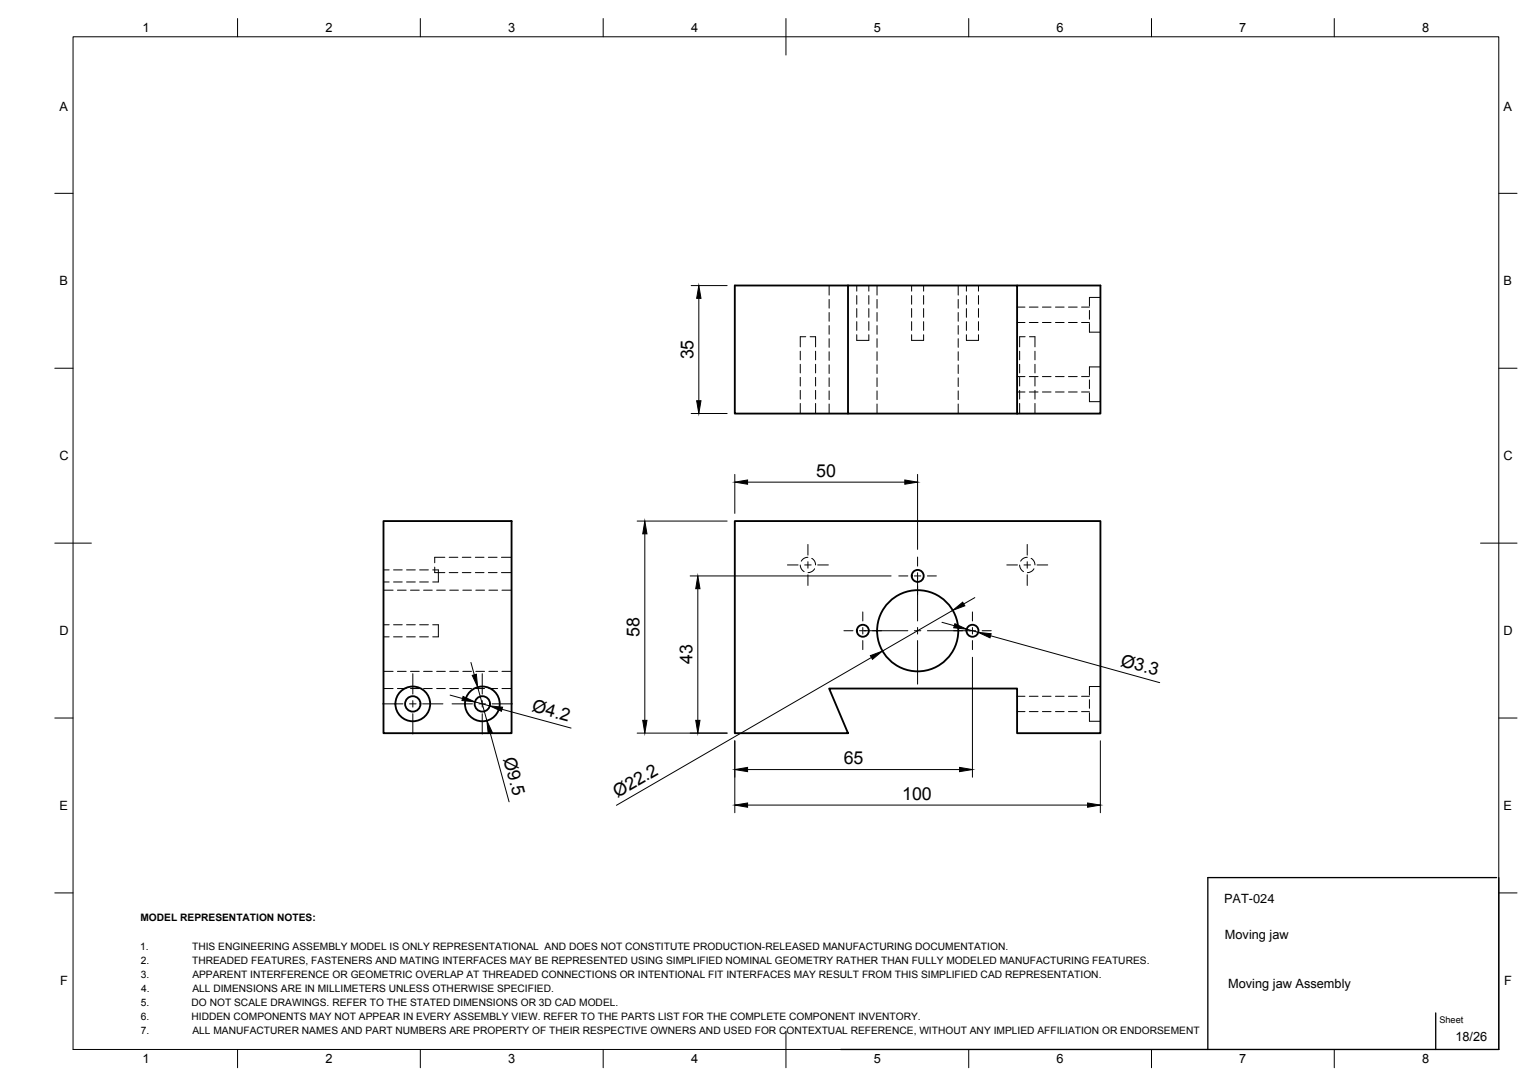
ISO-10303-21;
HEADER;
/* Generated by software containing ST-Developer
 * from STEP Tools, Inc. (www.steptools.com) 
 */

FILE_DESCRIPTION(
/* description */ ('Compact handwheel screw vise'),
/* implementation_level */ '2;1');

FILE_NAME(
/* name */ 'Moving jaw.step',
/* time_stamp */ '2026-10-29T16:08:22-07:00',
/* author */ (''),
/* organization */ (''),
/* preprocessor_version */ 'ST-DEVELOPER v20.2',
/* originating_system */ 'Autodesk Translation Framework v15.17.0.0',
/* authorisation */ '');

FILE_SCHEMA (('AUTOMOTIVE_DESIGN { 1 0 10303 214 3 1 1 }'));
ENDSEC;

DATA;
#10=MECHANICAL_DESIGN_GEOMETRIC_PRESENTATION_REPRESENTATION('',(#664),#25074);
#600=SHAPE_REPRESENTATION_RELATIONSHIP('SRR','None',#25210,#628);
#628=ADVANCED_BREP_SHAPE_REPRESENTATION('',(#699),#25057);
#664=STYLED_ITEM('',(#25432),#699);
#699=MANIFOLD_SOLID_BREP('Body1',#8073);
#769=FACE_BOUND('',#1695,.T.);
#770=FACE_BOUND('',#1699,.T.);
#771=FACE_BOUND('',#1703,.T.);
#772=FACE_BOUND('',#1704,.T.);
#773=FACE_BOUND('',#1708,.T.);
#774=FACE_BOUND('',#1709,.T.);
#775=FACE_BOUND('',#1710,.T.);
#776=FACE_BOUND('',#1711,.T.);
#777=FACE_BOUND('',#1714,.T.);
#778=FACE_BOUND('',#1715,.T.);
#779=FACE_BOUND('',#1718,.T.);
#780=FACE_BOUND('',#1719,.T.);
#781=FACE_BOUND('',#1720,.T.);
#896=PLANE('',#8711);
#897=PLANE('',#8715);
#898=PLANE('',#8719);
#899=PLANE('',#8723);
#900=PLANE('',#8727);
#901=PLANE('',#8731);
#902=PLANE('',#8738);
#903=PLANE('',#8745);
#904=PLANE('',#8746);
#905=PLANE('',#8747);
#906=PLANE('',#8748);
#907=PLANE('',#8749);
#908=PLANE('',#8750);
#909=PLANE('',#8751);
#910=PLANE('',#8752);
#911=PLANE('',#8753);
#912=PLANE('',#8754);
#1156=FACE_OUTER_BOUND('',#1683,.T.);
#1157=FACE_OUTER_BOUND('',#1684,.T.);
#1158=FACE_OUTER_BOUND('',#1685,.T.);
#1159=FACE_OUTER_BOUND('',#1686,.T.);
#1160=FACE_OUTER_BOUND('',#1687,.T.);
#1161=FACE_OUTER_BOUND('',#1688,.T.);
#1162=FACE_OUTER_BOUND('',#1689,.T.);
#1163=FACE_OUTER_BOUND('',#1690,.T.);
#1164=FACE_OUTER_BOUND('',#1691,.T.);
#1165=FACE_OUTER_BOUND('',#1692,.T.);
#1166=FACE_OUTER_BOUND('',#1693,.T.);
#1167=FACE_OUTER_BOUND('',#1694,.T.);
#1168=FACE_OUTER_BOUND('',#1696,.T.);
#1169=FACE_OUTER_BOUND('',#1697,.T.);
#1170=FACE_OUTER_BOUND('',#1698,.T.);
#1171=FACE_OUTER_BOUND('',#1700,.T.);
#1172=FACE_OUTER_BOUND('',#1701,.T.);
#1173=FACE_OUTER_BOUND('',#1702,.T.);
#1174=FACE_OUTER_BOUND('',#1705,.T.);
#1175=FACE_OUTER_BOUND('',#1706,.T.);
#1176=FACE_OUTER_BOUND('',#1707,.T.);
#1177=FACE_OUTER_BOUND('',#1712,.T.);
#1178=FACE_OUTER_BOUND('',#1713,.T.);
#1179=FACE_OUTER_BOUND('',#1716,.T.);
#1180=FACE_OUTER_BOUND('',#1717,.T.);
#1181=FACE_OUTER_BOUND('',#1721,.T.);
#1182=FACE_OUTER_BOUND('',#1722,.T.);
#1683=EDGE_LOOP('',(#5743,#5744,#5745,#5746));
#1684=EDGE_LOOP('',(#5747));
#1685=EDGE_LOOP('',(#5748,#5749,#5750,#5751));
#1686=EDGE_LOOP('',(#5752));
#1687=EDGE_LOOP('',(#5753,#5754,#5755,#5756));
#1688=EDGE_LOOP('',(#5757));
#1689=EDGE_LOOP('',(#5758,#5759,#5760,#5761));
#1690=EDGE_LOOP('',(#5762));
#1691=EDGE_LOOP('',(#5763,#5764,#5765,#5766));
#1692=EDGE_LOOP('',(#5767));
#1693=EDGE_LOOP('',(#5768,#5769,#5770,#5771));
#1694=EDGE_LOOP('',(#5772));
#1695=EDGE_LOOP('',(#5773));
#1696=EDGE_LOOP('',(#5774,#5775,#5776,#5777));
#1697=EDGE_LOOP('',(#5778,#5779,#5780,#5781));
#1698=EDGE_LOOP('',(#5782));
#1699=EDGE_LOOP('',(#5783));
#1700=EDGE_LOOP('',(#5784,#5785,#5786,#5787));
#1701=EDGE_LOOP('',(#5788,#5789,#5790,#5791));
#1702=EDGE_LOOP('',(#5792,#5793,#5794,#5795));
#1703=EDGE_LOOP('',(#5796));
#1704=EDGE_LOOP('',(#5797));
#1705=EDGE_LOOP('',(#5798,#5799,#5800,#5801));
#1706=EDGE_LOOP('',(#5802,#5803,#5804,#5805));
#1707=EDGE_LOOP('',(#5806,#5807,#5808,#5809,#5810,#5811,#5812,#5813));
#1708=EDGE_LOOP('',(#5814));
#1709=EDGE_LOOP('',(#5815));
#1710=EDGE_LOOP('',(#5816));
#1711=EDGE_LOOP('',(#5817));
#1712=EDGE_LOOP('',(#5818,#5819,#5820,#5821));
#1713=EDGE_LOOP('',(#5822,#5823,#5824,#5825));
#1714=EDGE_LOOP('',(#5826));
#1715=EDGE_LOOP('',(#5827));
#1716=EDGE_LOOP('',(#5828,#5829,#5830,#5831));
#1717=EDGE_LOOP('',(#5832,#5833,#5834,#5835,#5836,#5837,#5838,#5839));
#1718=EDGE_LOOP('',(#5840));
#1719=EDGE_LOOP('',(#5841));
#1720=EDGE_LOOP('',(#5842));
#1721=EDGE_LOOP('',(#5843,#5844,#5845,#5846));
#1722=EDGE_LOOP('',(#5847,#5848,#5849,#5850));
#2195=LINE('',#12321,#2703);
#2196=LINE('',#12328,#2704);
#2197=LINE('',#12335,#2705);
#2198=LINE('',#12342,#2706);
#2199=LINE('',#12349,#2707);
#2200=LINE('',#12356,#2708);
#2201=LINE('',#12364,#2709);
#2202=LINE('',#12369,#2710);
#2203=LINE('',#12377,#2711);
#2204=LINE('',#12382,#2712);
#2205=LINE('',#12387,#2713);
#2206=LINE('',#12389,#2714);
#2207=LINE('',#12391,#2715);
#2208=LINE('',#12392,#2716);
#2209=LINE('',#12395,#2717);
#2210=LINE('',#12397,#2718);
#2211=LINE('',#12398,#2719);
#2212=LINE('',#12401,#2720);
#2213=LINE('',#12403,#2721);
#2214=LINE('',#12404,#2722);
#2215=LINE('',#12407,#2723);
#2216=LINE('',#12409,#2724);
#2217=LINE('',#12411,#2725);
#2218=LINE('',#12413,#2726);
#2219=LINE('',#12414,#2727);
#2220=LINE('',#12417,#2728);
#2221=LINE('',#12418,#2729);
#2222=LINE('',#12421,#2730);
#2223=LINE('',#12422,#2731);
#2224=LINE('',#12425,#2732);
#2225=LINE('',#12427,#2733);
#2226=LINE('',#12428,#2734);
#2227=LINE('',#12430,#2735);
#2228=LINE('',#12431,#2736);
#2703=VECTOR('',#9955,0.165);
#2704=VECTOR('',#9964,0.165);
#2705=VECTOR('',#9973,0.165);
#2706=VECTOR('',#9982,0.21);
#2707=VECTOR('',#9991,0.21);
#2708=VECTOR('',#10000,0.475);
#2709=VECTOR('',#10011,0.210000000000001);
#2710=VECTOR('',#10016,0.475);
#2711=VECTOR('',#10027,0.210000000000001);
#2712=VECTOR('',#10032,1.11);
#2713=VECTOR('',#10037,1.);
#2714=VECTOR('',#10038,1.);
#2715=VECTOR('',#10039,1.);
#2716=VECTOR('',#10040,1.);
#2717=VECTOR('',#10043,1.);
#2718=VECTOR('',#10044,1.);
#2719=VECTOR('',#10045,1.);
#2720=VECTOR('',#10048,1.);
#2721=VECTOR('',#10049,1.);
#2722=VECTOR('',#10050,1.);
#2723=VECTOR('',#10053,1.);
#2724=VECTOR('',#10054,1.);
#2725=VECTOR('',#10055,1.);
#2726=VECTOR('',#10056,1.);
#2727=VECTOR('',#10057,1.);
#2728=VECTOR('',#10060,1.);
#2729=VECTOR('',#10061,1.);
#2730=VECTOR('',#10064,1.);
#2731=VECTOR('',#10065,1.);
#2732=VECTOR('',#10068,1.);
#2733=VECTOR('',#10069,1.);
#2734=VECTOR('',#10070,1.);
#2735=VECTOR('',#10073,1.);
#2736=VECTOR('',#10074,1.);
#3219=CIRCLE('',#8709,0.165);
#3220=CIRCLE('',#8710,0.165);
#3221=CIRCLE('',#8713,0.165);
#3222=CIRCLE('',#8714,0.165);
#3223=CIRCLE('',#8717,0.165);
#3224=CIRCLE('',#8718,0.165);
#3225=CIRCLE('',#8721,0.21);
#3226=CIRCLE('',#8722,0.21);
#3227=CIRCLE('',#8725,0.21);
#3228=CIRCLE('',#8726,0.21);
#3229=CIRCLE('',#8729,0.475);
#3230=CIRCLE('',#8730,0.475);
#3231=CIRCLE('',#8732,0.210000000000001);
#3232=CIRCLE('',#8734,0.210000000000001);
#3233=CIRCLE('',#8736,0.475);
#3234=CIRCLE('',#8737,0.475);
#3235=CIRCLE('',#8739,0.210000000000001);
#3236=CIRCLE('',#8741,0.210000000000001);
#3237=CIRCLE('',#8743,1.11);
#3238=CIRCLE('',#8744,1.11);
#3536=VERTEX_POINT('',#12318);
#3537=VERTEX_POINT('',#12320);
#3538=VERTEX_POINT('',#12325);
#3539=VERTEX_POINT('',#12327);
#3540=VERTEX_POINT('',#12332);
#3541=VERTEX_POINT('',#12334);
#3542=VERTEX_POINT('',#12339);
#3543=VERTEX_POINT('',#12341);
#3544=VERTEX_POINT('',#12346);
#3545=VERTEX_POINT('',#12348);
#3546=VERTEX_POINT('',#12353);
#3547=VERTEX_POINT('',#12355);
#3548=VERTEX_POINT('',#12359);
#3549=VERTEX_POINT('',#12362);
#3550=VERTEX_POINT('',#12366);
#3551=VERTEX_POINT('',#12368);
#3552=VERTEX_POINT('',#12372);
#3553=VERTEX_POINT('',#12375);
#3554=VERTEX_POINT('',#12379);
#3555=VERTEX_POINT('',#12381);
#3556=VERTEX_POINT('',#12385);
#3557=VERTEX_POINT('',#12386);
#3558=VERTEX_POINT('',#12388);
#3559=VERTEX_POINT('',#12390);
#3560=VERTEX_POINT('',#12394);
#3561=VERTEX_POINT('',#12396);
#3562=VERTEX_POINT('',#12400);
#3563=VERTEX_POINT('',#12402);
#3564=VERTEX_POINT('',#12406);
#3565=VERTEX_POINT('',#12408);
#3566=VERTEX_POINT('',#12410);
#3567=VERTEX_POINT('',#12412);
#3568=VERTEX_POINT('',#12416);
#3569=VERTEX_POINT('',#12420);
#3570=VERTEX_POINT('',#12424);
#3571=VERTEX_POINT('',#12426);
#4358=EDGE_CURVE('',#3536,#3536,#3219,.T.);
#4359=EDGE_CURVE('',#3536,#3537,#2195,.T.);
#4360=EDGE_CURVE('',#3537,#3537,#3220,.T.);
#4361=EDGE_CURVE('',#3538,#3538,#3221,.T.);
#4362=EDGE_CURVE('',#3538,#3539,#2196,.T.);
#4363=EDGE_CURVE('',#3539,#3539,#3222,.T.);
#4364=EDGE_CURVE('',#3540,#3540,#3223,.T.);
#4365=EDGE_CURVE('',#3540,#3541,#2197,.T.);
#4366=EDGE_CURVE('',#3541,#3541,#3224,.T.);
#4367=EDGE_CURVE('',#3542,#3542,#3225,.T.);
#4368=EDGE_CURVE('',#3542,#3543,#2198,.T.);
#4369=EDGE_CURVE('',#3543,#3543,#3226,.T.);
#4370=EDGE_CURVE('',#3544,#3544,#3227,.T.);
#4371=EDGE_CURVE('',#3544,#3545,#2199,.T.);
#4372=EDGE_CURVE('',#3545,#3545,#3228,.T.);
#4373=EDGE_CURVE('',#3546,#3546,#3229,.T.);
#4374=EDGE_CURVE('',#3546,#3547,#2200,.T.);
#4375=EDGE_CURVE('',#3547,#3547,#3230,.T.);
#4376=EDGE_CURVE('',#3548,#3548,#3231,.T.);
#4377=EDGE_CURVE('',#3549,#3549,#3232,.T.);
#4378=EDGE_CURVE('',#3549,#3548,#2201,.T.);
#4379=EDGE_CURVE('',#3550,#3550,#3233,.T.);
#4380=EDGE_CURVE('',#3550,#3551,#2202,.T.);
#4381=EDGE_CURVE('',#3551,#3551,#3234,.T.);
#4382=EDGE_CURVE('',#3552,#3552,#3235,.T.);
#4383=EDGE_CURVE('',#3553,#3553,#3236,.T.);
#4384=EDGE_CURVE('',#3553,#3552,#2203,.T.);
#4385=EDGE_CURVE('',#3554,#3554,#3237,.T.);
#4386=EDGE_CURVE('',#3554,#3555,#2204,.T.);
#4387=EDGE_CURVE('',#3555,#3555,#3238,.T.);
#4388=EDGE_CURVE('',#3556,#3557,#2205,.T.);
#4389=EDGE_CURVE('',#3558,#3556,#2206,.T.);
#4390=EDGE_CURVE('',#3559,#3558,#2207,.T.);
#4391=EDGE_CURVE('',#3557,#3559,#2208,.T.);
#4392=EDGE_CURVE('',#3560,#3556,#2209,.T.);
#4393=EDGE_CURVE('',#3561,#3560,#2210,.T.);
#4394=EDGE_CURVE('',#3558,#3561,#2211,.T.);
#4395=EDGE_CURVE('',#3562,#3560,#2212,.T.);
#4396=EDGE_CURVE('',#3563,#3562,#2213,.T.);
#4397=EDGE_CURVE('',#3561,#3563,#2214,.T.);
#4398=EDGE_CURVE('',#3557,#3564,#2215,.T.);
#4399=EDGE_CURVE('',#3564,#3565,#2216,.T.);
#4400=EDGE_CURVE('',#3566,#3565,#2217,.T.);
#4401=EDGE_CURVE('',#3567,#3566,#2218,.T.);
#4402=EDGE_CURVE('',#3567,#3562,#2219,.T.);
#4403=EDGE_CURVE('',#3568,#3559,#2220,.T.);
#4404=EDGE_CURVE('',#3564,#3568,#2221,.T.);
#4405=EDGE_CURVE('',#3568,#3569,#2222,.T.);
#4406=EDGE_CURVE('',#3565,#3569,#2223,.T.);
#4407=EDGE_CURVE('',#3570,#3567,#2224,.T.);
#4408=EDGE_CURVE('',#3571,#3566,#2225,.T.);
#4409=EDGE_CURVE('',#3570,#3571,#2226,.T.);
#4410=EDGE_CURVE('',#3563,#3570,#2227,.T.);
#4411=EDGE_CURVE('',#3569,#3571,#2228,.T.);
#5743=ORIENTED_EDGE('',*,*,#4358,.F.);
#5744=ORIENTED_EDGE('',*,*,#4359,.T.);
#5745=ORIENTED_EDGE('',*,*,#4360,.F.);
#5746=ORIENTED_EDGE('',*,*,#4359,.F.);
#5747=ORIENTED_EDGE('',*,*,#4358,.T.);
#5748=ORIENTED_EDGE('',*,*,#4361,.F.);
#5749=ORIENTED_EDGE('',*,*,#4362,.T.);
#5750=ORIENTED_EDGE('',*,*,#4363,.F.);
#5751=ORIENTED_EDGE('',*,*,#4362,.F.);
#5752=ORIENTED_EDGE('',*,*,#4361,.T.);
#5753=ORIENTED_EDGE('',*,*,#4364,.F.);
#5754=ORIENTED_EDGE('',*,*,#4365,.T.);
#5755=ORIENTED_EDGE('',*,*,#4366,.F.);
#5756=ORIENTED_EDGE('',*,*,#4365,.F.);
#5757=ORIENTED_EDGE('',*,*,#4364,.T.);
#5758=ORIENTED_EDGE('',*,*,#4367,.F.);
#5759=ORIENTED_EDGE('',*,*,#4368,.T.);
#5760=ORIENTED_EDGE('',*,*,#4369,.T.);
#5761=ORIENTED_EDGE('',*,*,#4368,.F.);
#5762=ORIENTED_EDGE('',*,*,#4369,.F.);
#5763=ORIENTED_EDGE('',*,*,#4370,.F.);
#5764=ORIENTED_EDGE('',*,*,#4371,.T.);
#5765=ORIENTED_EDGE('',*,*,#4372,.T.);
#5766=ORIENTED_EDGE('',*,*,#4371,.F.);
#5767=ORIENTED_EDGE('',*,*,#4372,.F.);
#5768=ORIENTED_EDGE('',*,*,#4373,.F.);
#5769=ORIENTED_EDGE('',*,*,#4374,.T.);
#5770=ORIENTED_EDGE('',*,*,#4375,.F.);
#5771=ORIENTED_EDGE('',*,*,#4374,.F.);
#5772=ORIENTED_EDGE('',*,*,#4373,.T.);
#5773=ORIENTED_EDGE('',*,*,#4376,.F.);
#5774=ORIENTED_EDGE('',*,*,#4377,.F.);
#5775=ORIENTED_EDGE('',*,*,#4378,.T.);
#5776=ORIENTED_EDGE('',*,*,#4376,.T.);
#5777=ORIENTED_EDGE('',*,*,#4378,.F.);
#5778=ORIENTED_EDGE('',*,*,#4379,.F.);
#5779=ORIENTED_EDGE('',*,*,#4380,.T.);
#5780=ORIENTED_EDGE('',*,*,#4381,.F.);
#5781=ORIENTED_EDGE('',*,*,#4380,.F.);
#5782=ORIENTED_EDGE('',*,*,#4379,.T.);
#5783=ORIENTED_EDGE('',*,*,#4382,.F.);
#5784=ORIENTED_EDGE('',*,*,#4383,.F.);
#5785=ORIENTED_EDGE('',*,*,#4384,.T.);
#5786=ORIENTED_EDGE('',*,*,#4382,.T.);
#5787=ORIENTED_EDGE('',*,*,#4384,.F.);
#5788=ORIENTED_EDGE('',*,*,#4385,.F.);
#5789=ORIENTED_EDGE('',*,*,#4386,.T.);
#5790=ORIENTED_EDGE('',*,*,#4387,.F.);
#5791=ORIENTED_EDGE('',*,*,#4386,.F.);
#5792=ORIENTED_EDGE('',*,*,#4388,.F.);
#5793=ORIENTED_EDGE('',*,*,#4389,.F.);
#5794=ORIENTED_EDGE('',*,*,#4390,.F.);
#5795=ORIENTED_EDGE('',*,*,#4391,.F.);
#5796=ORIENTED_EDGE('',*,*,#4377,.T.);
#5797=ORIENTED_EDGE('',*,*,#4383,.T.);
#5798=ORIENTED_EDGE('',*,*,#4392,.F.);
#5799=ORIENTED_EDGE('',*,*,#4393,.F.);
#5800=ORIENTED_EDGE('',*,*,#4394,.F.);
#5801=ORIENTED_EDGE('',*,*,#4389,.T.);
#5802=ORIENTED_EDGE('',*,*,#4395,.F.);
#5803=ORIENTED_EDGE('',*,*,#4396,.F.);
#5804=ORIENTED_EDGE('',*,*,#4397,.F.);
#5805=ORIENTED_EDGE('',*,*,#4393,.T.);
#5806=ORIENTED_EDGE('',*,*,#4395,.T.);
#5807=ORIENTED_EDGE('',*,*,#4392,.T.);
#5808=ORIENTED_EDGE('',*,*,#4388,.T.);
#5809=ORIENTED_EDGE('',*,*,#4398,.T.);
#5810=ORIENTED_EDGE('',*,*,#4399,.T.);
#5811=ORIENTED_EDGE('',*,*,#4400,.F.);
#5812=ORIENTED_EDGE('',*,*,#4401,.F.);
#5813=ORIENTED_EDGE('',*,*,#4402,.T.);
#5814=ORIENTED_EDGE('',*,*,#4360,.T.);
#5815=ORIENTED_EDGE('',*,*,#4363,.T.);
#5816=ORIENTED_EDGE('',*,*,#4366,.T.);
#5817=ORIENTED_EDGE('',*,*,#4387,.T.);
#5818=ORIENTED_EDGE('',*,*,#4391,.T.);
#5819=ORIENTED_EDGE('',*,*,#4403,.F.);
#5820=ORIENTED_EDGE('',*,*,#4404,.F.);
#5821=ORIENTED_EDGE('',*,*,#4398,.F.);
#5822=ORIENTED_EDGE('',*,*,#4404,.T.);
#5823=ORIENTED_EDGE('',*,*,#4405,.T.);
#5824=ORIENTED_EDGE('',*,*,#4406,.F.);
#5825=ORIENTED_EDGE('',*,*,#4399,.F.);
#5826=ORIENTED_EDGE('',*,*,#4375,.T.);
#5827=ORIENTED_EDGE('',*,*,#4381,.T.);
#5828=ORIENTED_EDGE('',*,*,#4407,.T.);
#5829=ORIENTED_EDGE('',*,*,#4401,.T.);
#5830=ORIENTED_EDGE('',*,*,#4408,.F.);
#5831=ORIENTED_EDGE('',*,*,#4409,.F.);
#5832=ORIENTED_EDGE('',*,*,#4397,.T.);
#5833=ORIENTED_EDGE('',*,*,#4410,.T.);
#5834=ORIENTED_EDGE('',*,*,#4409,.T.);
#5835=ORIENTED_EDGE('',*,*,#4411,.F.);
#5836=ORIENTED_EDGE('',*,*,#4405,.F.);
#5837=ORIENTED_EDGE('',*,*,#4403,.T.);
#5838=ORIENTED_EDGE('',*,*,#4390,.T.);
#5839=ORIENTED_EDGE('',*,*,#4394,.T.);
#5840=ORIENTED_EDGE('',*,*,#4367,.T.);
#5841=ORIENTED_EDGE('',*,*,#4370,.T.);
#5842=ORIENTED_EDGE('',*,*,#4385,.T.);
#5843=ORIENTED_EDGE('',*,*,#4411,.T.);
#5844=ORIENTED_EDGE('',*,*,#4408,.T.);
#5845=ORIENTED_EDGE('',*,*,#4400,.T.);
#5846=ORIENTED_EDGE('',*,*,#4406,.T.);
#5847=ORIENTED_EDGE('',*,*,#4396,.T.);
#5848=ORIENTED_EDGE('',*,*,#4402,.F.);
#5849=ORIENTED_EDGE('',*,*,#4407,.F.);
#5850=ORIENTED_EDGE('',*,*,#4410,.F.);
#7390=CYLINDRICAL_SURFACE('',#8708,0.165);
#7391=CYLINDRICAL_SURFACE('',#8712,0.165);
#7392=CYLINDRICAL_SURFACE('',#8716,0.165);
#7393=CYLINDRICAL_SURFACE('',#8720,0.21);
#7394=CYLINDRICAL_SURFACE('',#8724,0.21);
#7395=CYLINDRICAL_SURFACE('',#8728,0.475);
#7396=CYLINDRICAL_SURFACE('',#8733,0.210000000000001);
#7397=CYLINDRICAL_SURFACE('',#8735,0.475);
#7398=CYLINDRICAL_SURFACE('',#8740,0.210000000000001);
#7399=CYLINDRICAL_SURFACE('',#8742,1.11);
#7726=ADVANCED_FACE('',(#1156),#7390,.F.);
#7727=ADVANCED_FACE('',(#1157),#896,.T.);
#7728=ADVANCED_FACE('',(#1158),#7391,.F.);
#7729=ADVANCED_FACE('',(#1159),#897,.T.);
#7730=ADVANCED_FACE('',(#1160),#7392,.F.);
#7731=ADVANCED_FACE('',(#1161),#898,.T.);
#7732=ADVANCED_FACE('',(#1162),#7393,.F.);
#7733=ADVANCED_FACE('',(#1163),#899,.F.);
#7734=ADVANCED_FACE('',(#1164),#7394,.F.);
#7735=ADVANCED_FACE('',(#1165),#900,.F.);
#7736=ADVANCED_FACE('',(#1166),#7395,.F.);
#7737=ADVANCED_FACE('',(#1167,#769),#901,.T.);
#7738=ADVANCED_FACE('',(#1168),#7396,.F.);
#7739=ADVANCED_FACE('',(#1169),#7397,.F.);
#7740=ADVANCED_FACE('',(#1170,#770),#902,.T.);
#7741=ADVANCED_FACE('',(#1171),#7398,.F.);
#7742=ADVANCED_FACE('',(#1172),#7399,.F.);
#7743=ADVANCED_FACE('',(#1173,#771,#772),#903,.F.);
#7744=ADVANCED_FACE('',(#1174),#904,.F.);
#7745=ADVANCED_FACE('',(#1175),#905,.F.);
#7746=ADVANCED_FACE('',(#1176,#773,#774,#775,#776),#906,.T.);
#7747=ADVANCED_FACE('',(#1177),#907,.F.);
#7748=ADVANCED_FACE('',(#1178,#777,#778),#908,.T.);
#7749=ADVANCED_FACE('',(#1179),#909,.T.);
#7750=ADVANCED_FACE('',(#1180,#779,#780,#781),#910,.T.);
#7751=ADVANCED_FACE('',(#1181),#911,.T.);
#7752=ADVANCED_FACE('',(#1182),#912,.F.);
#8073=CLOSED_SHELL('',(#7726,#7727,#7728,#7729,#7730,#7731,#7732,#7733,
#7734,#7735,#7736,#7737,#7738,#7739,#7740,#7741,#7742,#7743,#7744,#7745,
#7746,#7747,#7748,#7749,#7750,#7751,#7752));
#8707=AXIS2_PLACEMENT_3D('',#12316,#9949,#9950);
#8708=AXIS2_PLACEMENT_3D('',#12317,#9951,#9952);
#8709=AXIS2_PLACEMENT_3D('',#12319,#9953,#9954);
#8710=AXIS2_PLACEMENT_3D('',#12322,#9956,#9957);
#8711=AXIS2_PLACEMENT_3D('',#12323,#9958,#9959);
#8712=AXIS2_PLACEMENT_3D('',#12324,#9960,#9961);
#8713=AXIS2_PLACEMENT_3D('',#12326,#9962,#9963);
#8714=AXIS2_PLACEMENT_3D('',#12329,#9965,#9966);
#8715=AXIS2_PLACEMENT_3D('',#12330,#9967,#9968);
#8716=AXIS2_PLACEMENT_3D('',#12331,#9969,#9970);
#8717=AXIS2_PLACEMENT_3D('',#12333,#9971,#9972);
#8718=AXIS2_PLACEMENT_3D('',#12336,#9974,#9975);
#8719=AXIS2_PLACEMENT_3D('',#12337,#9976,#9977);
#8720=AXIS2_PLACEMENT_3D('',#12338,#9978,#9979);
#8721=AXIS2_PLACEMENT_3D('',#12340,#9980,#9981);
#8722=AXIS2_PLACEMENT_3D('',#12343,#9983,#9984);
#8723=AXIS2_PLACEMENT_3D('',#12344,#9985,#9986);
#8724=AXIS2_PLACEMENT_3D('',#12345,#9987,#9988);
#8725=AXIS2_PLACEMENT_3D('',#12347,#9989,#9990);
#8726=AXIS2_PLACEMENT_3D('',#12350,#9992,#9993);
#8727=AXIS2_PLACEMENT_3D('',#12351,#9994,#9995);
#8728=AXIS2_PLACEMENT_3D('',#12352,#9996,#9997);
#8729=AXIS2_PLACEMENT_3D('',#12354,#9998,#9999);
#8730=AXIS2_PLACEMENT_3D('',#12357,#10001,#10002);
#8731=AXIS2_PLACEMENT_3D('',#12358,#10003,#10004);
#8732=AXIS2_PLACEMENT_3D('',#12360,#10005,#10006);
#8733=AXIS2_PLACEMENT_3D('',#12361,#10007,#10008);
#8734=AXIS2_PLACEMENT_3D('',#12363,#10009,#10010);
#8735=AXIS2_PLACEMENT_3D('',#12365,#10012,#10013);
#8736=AXIS2_PLACEMENT_3D('',#12367,#10014,#10015);
#8737=AXIS2_PLACEMENT_3D('',#12370,#10017,#10018);
#8738=AXIS2_PLACEMENT_3D('',#12371,#10019,#10020);
#8739=AXIS2_PLACEMENT_3D('',#12373,#10021,#10022);
#8740=AXIS2_PLACEMENT_3D('',#12374,#10023,#10024);
#8741=AXIS2_PLACEMENT_3D('',#12376,#10025,#10026);
#8742=AXIS2_PLACEMENT_3D('',#12378,#10028,#10029);
#8743=AXIS2_PLACEMENT_3D('',#12380,#10030,#10031);
#8744=AXIS2_PLACEMENT_3D('',#12383,#10033,#10034);
#8745=AXIS2_PLACEMENT_3D('',#12384,#10035,#10036);
#8746=AXIS2_PLACEMENT_3D('',#12393,#10041,#10042);
#8747=AXIS2_PLACEMENT_3D('',#12399,#10046,#10047);
#8748=AXIS2_PLACEMENT_3D('',#12405,#10051,#10052);
#8749=AXIS2_PLACEMENT_3D('',#12415,#10058,#10059);
#8750=AXIS2_PLACEMENT_3D('',#12419,#10062,#10063);
#8751=AXIS2_PLACEMENT_3D('',#12423,#10066,#10067);
#8752=AXIS2_PLACEMENT_3D('',#12429,#10071,#10072);
#8753=AXIS2_PLACEMENT_3D('',#12432,#10075,#10076);
#8754=AXIS2_PLACEMENT_3D('',#12433,#10077,#10078);
#9949=DIRECTION('axis',(0.,0.,1.));
#9950=DIRECTION('refdir',(1.,0.,0.));
#9951=DIRECTION('center_axis',(1.,0.,0.));
#9952=DIRECTION('ref_axis',(0.,0.,-1.));
#9953=DIRECTION('center_axis',(1.,0.,0.));
#9954=DIRECTION('ref_axis',(0.,0.,-1.));
#9955=DIRECTION('',(1.,0.,0.));
#9956=DIRECTION('center_axis',(-1.,0.,0.));
#9957=DIRECTION('ref_axis',(0.,0.,-1.));
#9958=DIRECTION('center_axis',(1.,0.,0.));
#9959=DIRECTION('ref_axis',(0.,0.,-1.));
#9960=DIRECTION('center_axis',(1.,0.,0.));
#9961=DIRECTION('ref_axis',(0.,0.,-1.));
#9962=DIRECTION('center_axis',(1.,0.,0.));
#9963=DIRECTION('ref_axis',(0.,0.,-1.));
#9964=DIRECTION('',(1.,0.,0.));
#9965=DIRECTION('center_axis',(-1.,0.,0.));
#9966=DIRECTION('ref_axis',(0.,0.,-1.));
#9967=DIRECTION('center_axis',(1.,0.,0.));
#9968=DIRECTION('ref_axis',(0.,0.,-1.));
#9969=DIRECTION('center_axis',(1.,0.,0.));
#9970=DIRECTION('ref_axis',(0.,0.,-1.));
#9971=DIRECTION('center_axis',(1.,0.,0.));
#9972=DIRECTION('ref_axis',(0.,0.,-1.));
#9973=DIRECTION('',(1.,0.,0.));
#9974=DIRECTION('center_axis',(-1.,0.,0.));
#9975=DIRECTION('ref_axis',(0.,0.,-1.));
#9976=DIRECTION('center_axis',(1.,0.,0.));
#9977=DIRECTION('ref_axis',(0.,0.,-1.));
#9978=DIRECTION('center_axis',(1.,0.,0.));
#9979=DIRECTION('ref_axis',(0.,0.,-1.));
#9980=DIRECTION('center_axis',(1.,0.,0.));
#9981=DIRECTION('ref_axis',(0.,0.,-1.));
#9982=DIRECTION('',(1.,0.,0.));
#9983=DIRECTION('center_axis',(1.,0.,0.));
#9984=DIRECTION('ref_axis',(0.,0.,-1.));
#9985=DIRECTION('center_axis',(1.,0.,0.));
#9986=DIRECTION('ref_axis',(0.,0.,-1.));
#9987=DIRECTION('center_axis',(1.,0.,0.));
#9988=DIRECTION('ref_axis',(0.,0.,-1.));
#9989=DIRECTION('center_axis',(1.,0.,0.));
#9990=DIRECTION('ref_axis',(0.,0.,-1.));
#9991=DIRECTION('',(1.,0.,0.));
#9992=DIRECTION('center_axis',(1.,0.,0.));
#9993=DIRECTION('ref_axis',(0.,0.,-1.));
#9994=DIRECTION('center_axis',(1.,0.,0.));
#9995=DIRECTION('ref_axis',(0.,0.,-1.));
#9996=DIRECTION('center_axis',(0.,1.,0.));
#9997=DIRECTION('ref_axis',(1.,0.,0.));
#9998=DIRECTION('center_axis',(0.,1.,0.));
#9999=DIRECTION('ref_axis',(1.,0.,0.));
#10000=DIRECTION('',(0.,1.,0.));
#10001=DIRECTION('center_axis',(0.,-1.,0.));
#10002=DIRECTION('ref_axis',(1.,0.,0.));
#10003=DIRECTION('center_axis',(0.,1.,0.));
#10004=DIRECTION('ref_axis',(1.,0.,0.));
#10005=DIRECTION('center_axis',(0.,1.,0.));
#10006=DIRECTION('ref_axis',(1.,0.,0.));
#10007=DIRECTION('center_axis',(0.,1.,0.));
#10008=DIRECTION('ref_axis',(1.,0.,0.));
#10009=DIRECTION('center_axis',(0.,1.,0.));
#10010=DIRECTION('ref_axis',(1.,0.,0.));
#10011=DIRECTION('',(0.,1.,0.));
#10012=DIRECTION('center_axis',(0.,1.,0.));
#10013=DIRECTION('ref_axis',(1.,0.,0.));
#10014=DIRECTION('center_axis',(0.,1.,0.));
#10015=DIRECTION('ref_axis',(1.,0.,0.));
#10016=DIRECTION('',(0.,1.,0.));
#10017=DIRECTION('center_axis',(0.,-1.,0.));
#10018=DIRECTION('ref_axis',(1.,0.,0.));
#10019=DIRECTION('center_axis',(0.,1.,0.));
#10020=DIRECTION('ref_axis',(1.,0.,0.));
#10021=DIRECTION('center_axis',(0.,1.,0.));
#10022=DIRECTION('ref_axis',(1.,0.,0.));
#10023=DIRECTION('center_axis',(0.,1.,0.));
#10024=DIRECTION('ref_axis',(1.,0.,0.));
#10025=DIRECTION('center_axis',(0.,1.,0.));
#10026=DIRECTION('ref_axis',(1.,0.,0.));
#10027=DIRECTION('',(0.,1.,0.));
#10028=DIRECTION('center_axis',(1.,0.,0.));
#10029=DIRECTION('ref_axis',(0.,0.,-1.));
#10030=DIRECTION('center_axis',(1.,0.,0.));
#10031=DIRECTION('ref_axis',(0.,0.,-1.));
#10032=DIRECTION('',(1.,0.,0.));
#10033=DIRECTION('center_axis',(-1.,0.,0.));
#10034=DIRECTION('ref_axis',(0.,0.,-1.));
#10035=DIRECTION('center_axis',(0.,1.,0.));
#10036=DIRECTION('ref_axis',(0.,0.,1.));
#10037=DIRECTION('',(0.,0.,-1.));
#10038=DIRECTION('',(1.,0.,0.));
#10039=DIRECTION('',(0.,0.,1.));
#10040=DIRECTION('',(-1.,0.,0.));
#10041=DIRECTION('center_axis',(0.,0.,1.));
#10042=DIRECTION('ref_axis',(0.,-1.,0.));
#10043=DIRECTION('',(0.,1.,0.));
#10044=DIRECTION('',(1.,0.,0.));
#10045=DIRECTION('',(0.,-1.,0.));
#10046=DIRECTION('center_axis',(0.,-0.921146216293932,-0.389216711110112));
#10047=DIRECTION('ref_axis',(0.,0.389216711110112,-0.921146216293932));
#10048=DIRECTION('',(0.,-0.389216711110112,0.921146216293932));
#10049=DIRECTION('',(1.,0.,0.));
#10050=DIRECTION('',(0.,0.389216711110112,-0.921146216293932));
#10051=DIRECTION('center_axis',(1.,0.,0.));
#10052=DIRECTION('ref_axis',(0.,1.,0.));
#10053=DIRECTION('',(0.,1.,0.));
#10054=DIRECTION('',(0.,0.,1.));
#10055=DIRECTION('',(0.,1.,0.));
#10056=DIRECTION('',(0.,0.,1.));
#10057=DIRECTION('',(0.,1.,0.));
#10058=DIRECTION('center_axis',(0.,0.,1.));
#10059=DIRECTION('ref_axis',(1.,0.,0.));
#10060=DIRECTION('',(0.,-1.,0.));
#10061=DIRECTION('',(-1.,0.,0.));
#10062=DIRECTION('center_axis',(0.,1.,0.));
#10063=DIRECTION('ref_axis',(-1.,0.,0.));
#10064=DIRECTION('',(0.,0.,1.));
#10065=DIRECTION('',(-1.,0.,0.));
#10066=DIRECTION('center_axis',(0.,-1.,0.));
#10067=DIRECTION('ref_axis',(1.,0.,0.));
#10068=DIRECTION('',(1.,0.,0.));
#10069=DIRECTION('',(1.,0.,0.));
#10070=DIRECTION('',(0.,0.,1.));
#10071=DIRECTION('center_axis',(-1.,0.,0.));
#10072=DIRECTION('ref_axis',(0.,-1.,0.));
#10073=DIRECTION('',(0.,-1.,0.));
#10074=DIRECTION('',(0.,-1.,0.));
#10075=DIRECTION('center_axis',(0.,0.,1.));
#10076=DIRECTION('ref_axis',(1.,0.,0.));
#10077=DIRECTION('center_axis',(0.,0.,1.));
#10078=DIRECTION('ref_axis',(1.,0.,0.));
#12316=CARTESIAN_POINT('',(0.,0.,0.));
#12317=CARTESIAN_POINT('Origin',(13.,-1.5,4.));
#12318=CARTESIAN_POINT('',(13.,-1.5,4.165));
#12319=CARTESIAN_POINT('Origin',(13.,-1.5,4.));
#12320=CARTESIAN_POINT('',(14.5,-1.5,4.165));
#12321=CARTESIAN_POINT('',(13.,-1.5,4.165));
#12322=CARTESIAN_POINT('Origin',(14.5,-1.5,4.));
#12323=CARTESIAN_POINT('Origin',(13.,-1.5,4.));
#12324=CARTESIAN_POINT('Origin',(13.,1.5,4.));
#12325=CARTESIAN_POINT('',(13.,1.5,4.165));
#12326=CARTESIAN_POINT('Origin',(13.,1.5,4.));
#12327=CARTESIAN_POINT('',(14.5,1.5,4.165));
#12328=CARTESIAN_POINT('',(13.,1.5,4.165));
#12329=CARTESIAN_POINT('Origin',(14.5,1.5,4.));
#12330=CARTESIAN_POINT('Origin',(13.,1.5,4.));
#12331=CARTESIAN_POINT('Origin',(13.,0.,5.5));
#12332=CARTESIAN_POINT('',(13.,-2.02066721859313E-17,5.665));
#12333=CARTESIAN_POINT('Origin',(13.,0.,5.5));
#12334=CARTESIAN_POINT('',(14.5,2.02066721859313E-17,5.665));
#12335=CARTESIAN_POINT('',(13.,-2.02066721859313E-17,5.665));
#12336=CARTESIAN_POINT('Origin',(14.5,0.,5.5));
#12337=CARTESIAN_POINT('Origin',(13.,0.,5.5));
#12338=CARTESIAN_POINT('Origin',(10.9,-3.,5.8));
#12339=CARTESIAN_POINT('',(11.,-3.,6.01));
#12340=CARTESIAN_POINT('Origin',(11.,-3.,5.8));
#12341=CARTESIAN_POINT('',(13.1,-3.,6.01));
#12342=CARTESIAN_POINT('',(10.9,-3.,6.01));
#12343=CARTESIAN_POINT('Origin',(13.1,-3.,5.8));
#12344=CARTESIAN_POINT('Origin',(13.1,-3.,5.8));
#12345=CARTESIAN_POINT('Origin',(10.9,3.,5.8));
#12346=CARTESIAN_POINT('',(11.,3.,6.01));
#12347=CARTESIAN_POINT('Origin',(11.,3.,5.8));
#12348=CARTESIAN_POINT('',(13.1,3.,6.01));
#12349=CARTESIAN_POINT('',(10.9,3.,6.01));
#12350=CARTESIAN_POINT('Origin',(13.1,3.,5.8));
#12351=CARTESIAN_POINT('Origin',(13.1,3.,5.8));
#12352=CARTESIAN_POINT('Origin',(13.7,4.7,2.));
#12353=CARTESIAN_POINT('',(13.225,4.7,2.));
#12354=CARTESIAN_POINT('Origin',(13.7,4.7,2.));
#12355=CARTESIAN_POINT('',(13.225,5.,2.));
#12356=CARTESIAN_POINT('',(13.225,4.7,2.));
#12357=CARTESIAN_POINT('Origin',(13.7,5.,2.));
#12358=CARTESIAN_POINT('Origin',(13.7,4.7,2.));
#12359=CARTESIAN_POINT('',(13.49,4.7,2.));
#12360=CARTESIAN_POINT('Origin',(13.7,4.7,2.));
#12361=CARTESIAN_POINT('Origin',(13.7,2.72,2.));
#12362=CARTESIAN_POINT('',(13.49,2.72,2.));
#12363=CARTESIAN_POINT('Origin',(13.7,2.72,2.));
#12364=CARTESIAN_POINT('',(13.49,2.72,2.));
#12365=CARTESIAN_POINT('Origin',(11.8,4.7,2.));
#12366=CARTESIAN_POINT('',(11.325,4.7,2.));
#12367=CARTESIAN_POINT('Origin',(11.8,4.7,2.));
#12368=CARTESIAN_POINT('',(11.325,5.,2.));
#12369=CARTESIAN_POINT('',(11.325,4.7,2.));
#12370=CARTESIAN_POINT('Origin',(11.8,5.,2.));
#12371=CARTESIAN_POINT('Origin',(11.8,4.7,2.));
#12372=CARTESIAN_POINT('',(11.59,4.7,2.));
#12373=CARTESIAN_POINT('Origin',(11.8,4.7,2.));
#12374=CARTESIAN_POINT('Origin',(11.8,2.72,2.));
#12375=CARTESIAN_POINT('',(11.59,2.72,2.));
#12376=CARTESIAN_POINT('Origin',(11.8,2.72,2.));
#12377=CARTESIAN_POINT('',(11.59,2.72,2.));
#12378=CARTESIAN_POINT('Origin',(10.9,0.,4.));
#12379=CARTESIAN_POINT('',(11.,-1.35935794705356E-16,5.11));
#12380=CARTESIAN_POINT('Origin',(11.,0.,4.));
#12381=CARTESIAN_POINT('',(14.5,1.35935794705356E-16,5.11));
#12382=CARTESIAN_POINT('',(10.9,-1.35935794705356E-16,5.11));
#12383=CARTESIAN_POINT('Origin',(14.5,0.,4.));
#12384=CARTESIAN_POINT('Origin',(10.9,2.72,1.));
#12385=CARTESIAN_POINT('',(14.5,2.72,2.42));
#12386=CARTESIAN_POINT('',(14.5,2.72,1.2));
#12387=CARTESIAN_POINT('',(14.5,2.72,1.1));
#12388=CARTESIAN_POINT('',(11.,2.72,2.42));
#12389=CARTESIAN_POINT('',(10.9,2.72,2.42));
#12390=CARTESIAN_POINT('',(11.,2.72,1.2));
#12391=CARTESIAN_POINT('',(11.,2.72,1.1));
#12392=CARTESIAN_POINT('',(11.825,2.72,1.2));
#12393=CARTESIAN_POINT('Origin',(10.9,2.72,2.42));
#12394=CARTESIAN_POINT('',(14.5,-2.42,2.42));
#12395=CARTESIAN_POINT('',(14.5,-1.14,2.42));
#12396=CARTESIAN_POINT('',(11.,-2.42,2.42));
#12397=CARTESIAN_POINT('',(10.9,-2.42,2.42));
#12398=CARTESIAN_POINT('',(11.,3.86,2.42));
#12399=CARTESIAN_POINT('Origin',(10.9,-2.42,2.42));
#12400=CARTESIAN_POINT('',(14.5,-1.90450704225352,1.2));
#12401=CARTESIAN_POINT('',(14.5,-2.39672109072547,2.36490658138361));
#12402=CARTESIAN_POINT('',(11.,-1.90450704225352,1.2));
#12403=CARTESIAN_POINT('',(11.825,-1.90450704225352,1.2));
#12404=CARTESIAN_POINT('',(11.,-1.6392728496886,0.572279077596364));
#12405=CARTESIAN_POINT('Origin',(14.5,-5.,1.2));
#12406=CARTESIAN_POINT('',(14.5,5.,1.2));
#12407=CARTESIAN_POINT('',(14.5,-5.,1.2));
#12408=CARTESIAN_POINT('',(14.5,5.,7.));
#12409=CARTESIAN_POINT('',(14.5,5.,1.2));
#12410=CARTESIAN_POINT('',(14.5,-5.,7.));
#12411=CARTESIAN_POINT('',(14.5,-5.,7.));
#12412=CARTESIAN_POINT('',(14.5,-5.,1.2));
#12413=CARTESIAN_POINT('',(14.5,-5.,1.2));
#12414=CARTESIAN_POINT('',(14.5,-5.,1.2));
#12415=CARTESIAN_POINT('Origin',(12.75,0.,1.2));
#12416=CARTESIAN_POINT('',(11.,5.,1.2));
#12417=CARTESIAN_POINT('',(11.,5.,1.2));
#12418=CARTESIAN_POINT('',(14.5,5.,1.2));
#12419=CARTESIAN_POINT('Origin',(14.5,5.,1.2));
#12420=CARTESIAN_POINT('',(11.,5.,7.));
#12421=CARTESIAN_POINT('',(11.,5.,1.2));
#12422=CARTESIAN_POINT('',(14.5,5.,7.));
#12423=CARTESIAN_POINT('Origin',(11.,-5.,1.2));
#12424=CARTESIAN_POINT('',(11.,-5.,1.2));
#12425=CARTESIAN_POINT('',(11.,-5.,1.2));
#12426=CARTESIAN_POINT('',(11.,-5.,7.));
#12427=CARTESIAN_POINT('',(11.,-5.,7.));
#12428=CARTESIAN_POINT('',(11.,-5.,1.2));
#12429=CARTESIAN_POINT('Origin',(11.,5.,1.2));
#12430=CARTESIAN_POINT('',(11.,5.,1.2));
#12431=CARTESIAN_POINT('',(11.,5.,7.));
#12432=CARTESIAN_POINT('Origin',(12.75,0.,7.));
#12433=CARTESIAN_POINT('Origin',(12.75,0.,1.2));
#25023=UNCERTAINTY_MEASURE_WITH_UNIT(LENGTH_MEASURE(0.001),#25075,
'DISTANCE_ACCURACY_VALUE',
'Maximum model space distance between geometric entities at asserted c
onnectivities');
#25040=UNCERTAINTY_MEASURE_WITH_UNIT(LENGTH_MEASURE(0.001),#25075,
'DISTANCE_ACCURACY_VALUE',
'Maximum model space distance between geometric entities at asserted c
onnectivities');
#25057=(
GEOMETRIC_REPRESENTATION_CONTEXT(3)
GLOBAL_UNCERTAINTY_ASSIGNED_CONTEXT((#25023))
GLOBAL_UNIT_ASSIGNED_CONTEXT((#25075,#25077,#25078))
REPRESENTATION_CONTEXT('','3D')
);
#25074=(
GEOMETRIC_REPRESENTATION_CONTEXT(3)
GLOBAL_UNCERTAINTY_ASSIGNED_CONTEXT((#25040))
GLOBAL_UNIT_ASSIGNED_CONTEXT((#25075,#25077,#25078))
REPRESENTATION_CONTEXT('','3D')
);
#25075=(
LENGTH_UNIT()
NAMED_UNIT(*)
SI_UNIT(.CENTI.,.METRE.)
);
#25077=(
NAMED_UNIT(*)
PLANE_ANGLE_UNIT()
SI_UNIT($,.RADIAN.)
);
#25078=(
NAMED_UNIT(*)
SI_UNIT($,.STERADIAN.)
SOLID_ANGLE_UNIT()
);
#25095=SHAPE_DEFINITION_REPRESENTATION(#25133,#25210);
#25133=PRODUCT_DEFINITION_SHAPE('',$,#25244);
#25210=SHAPE_REPRESENTATION('',(#8707),#25057);
#25227=PRODUCT_DEFINITION_CONTEXT('part definition',#25328,'design');
#25244=PRODUCT_DEFINITION('Moving jaw','Moving jaw',#25277,#25227);
#25277=PRODUCT_DEFINITION_FORMATION('',$,#25346);
#25328=APPLICATION_CONTEXT(
'Core Data for Automotive Mechanical Design Process');
#25329=PRODUCT_CONTEXT('part definition',#25328,'mechanical');
#25346=PRODUCT('Moving jaw','Moving jaw','Moving jaw',(#25329));
#25426=COLOUR_RGB('Sky Blue',0.24,0.69,0.87);
#25427=FILL_AREA_STYLE_COLOUR('',#25426);
#25428=FILL_AREA_STYLE('',(#25427));
#25429=SURFACE_STYLE_FILL_AREA(#25428);
#25430=SURFACE_SIDE_STYLE('',(#25429));
#25431=SURFACE_STYLE_USAGE(.BOTH.,#25430);
#25432=PRESENTATION_STYLE_ASSIGNMENT((#25431));
ENDSEC;
END-ISO-10303-21;
